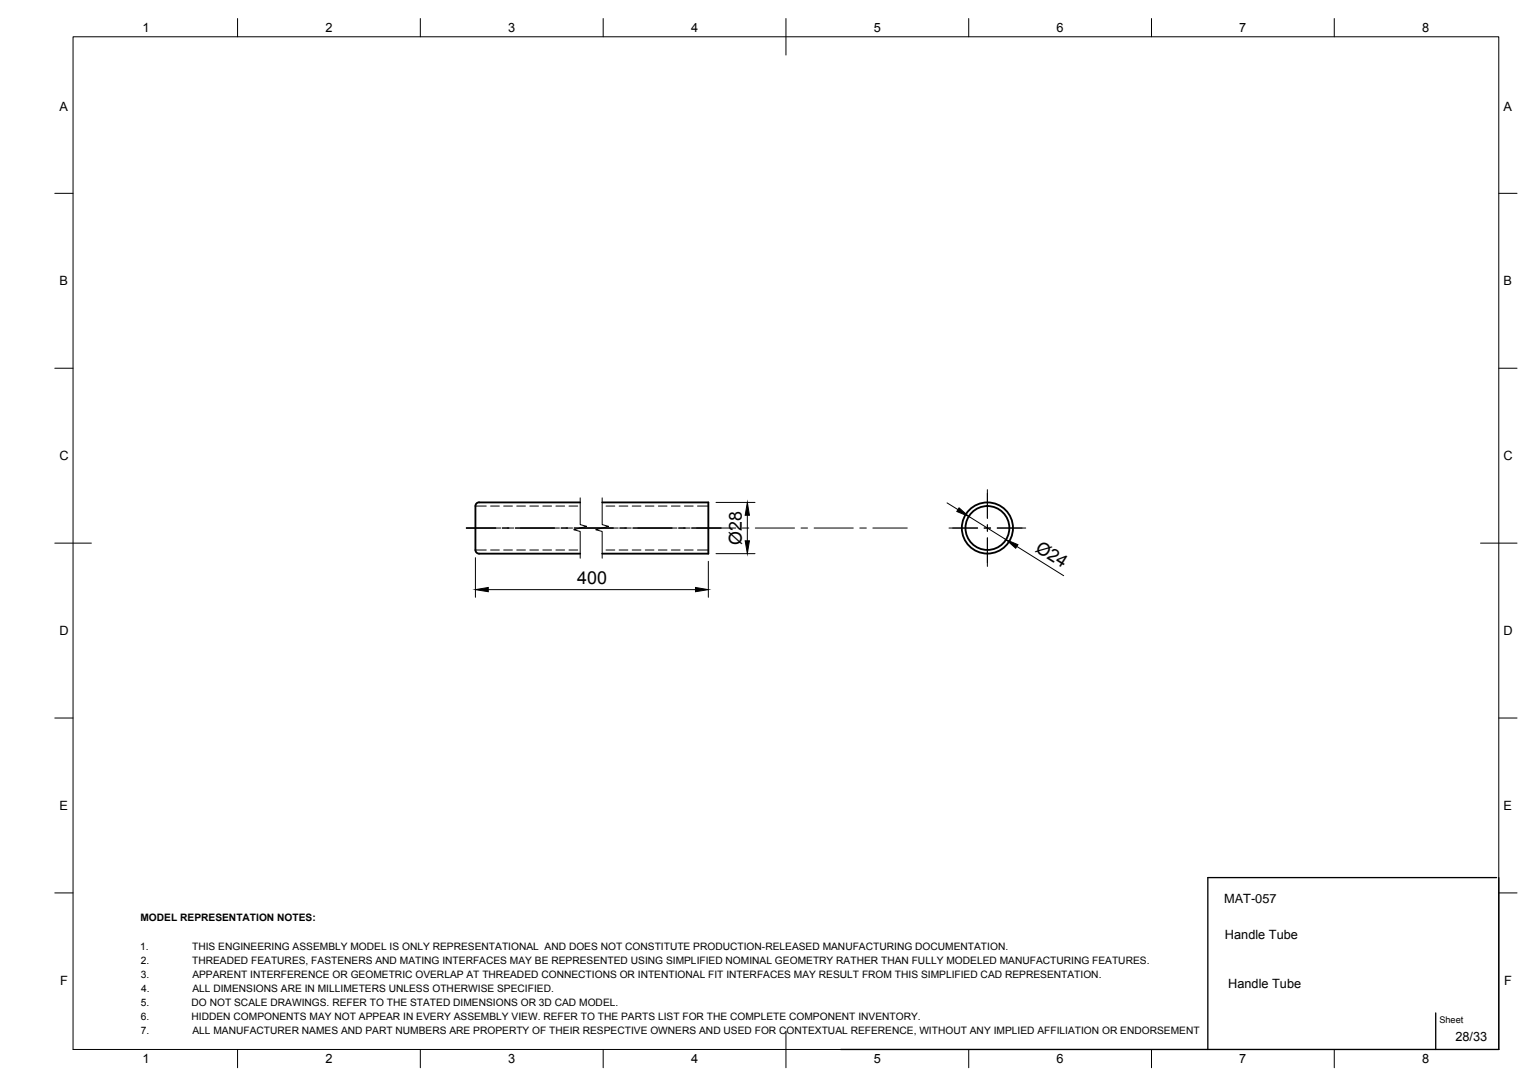
ISO-10303-21;
HEADER;
/* Generated by software containing ST-Developer
 * from STEP Tools, Inc. (www.steptools.com) 
 */

FILE_DESCRIPTION(
/* description */ ('STEP AP214', 'CAx-IF Rec.Pracs.---Representation and Presentation of Product Manufa
cturing Information (PMI)---4.0---2014-10-13'),
/* implementation_level */ '2;1');

FILE_NAME(
/* name */ 'Handle Tube.step',
/* time_stamp */ '2026-10-28T23:34:22+01:00',
/* author */ (''),
/* organization */ (''),
/* preprocessor_version */ 'ST-DEVELOPER v20.2',
/* originating_system */ 'Autodesk Translation Framework v15.17.0.0',
/* authorisation */ '');

FILE_SCHEMA (('AP242_MANAGED_MODEL_BASED_3D_ENGINEERING_MIM_LF { 1 0 10303 442 2 1 4 }'));
ENDSEC;

DATA;
#10=MECHANICAL_DESIGN_GEOMETRIC_PRESENTATION_REPRESENTATION('',(#269),#27807);
#221=SHAPE_REPRESENTATION_RELATIONSHIP('SRR','None',#27919,#243);
#243=ADVANCED_BREP_SHAPE_REPRESENTATION('',(#298),#27799);
#269=STYLED_ITEM('',(#28063),#298);
#298=MANIFOLD_SOLID_BREP('Body1',#12045);
#425=FACE_BOUND('',#2573,.T.);
#689=PLANE('',#13433);
#839=TOROIDAL_SURFACE('',#13423,12.,2.);
#1175=CYLINDRICAL_SURFACE('',#13429,12.);
#1176=CYLINDRICAL_SURFACE('',#13431,14.);
#1782=FACE_OUTER_BOUND('',#2569,.T.);
#1783=FACE_OUTER_BOUND('',#2570,.T.);
#1784=FACE_OUTER_BOUND('',#2571,.T.);
#1785=FACE_OUTER_BOUND('',#2572,.T.);
#2569=EDGE_LOOP('',(#10521,#10522,#10523,#10524,#10525,#10526));
#2570=EDGE_LOOP('',(#10527,#10528,#10529,#10530,#10531));
#2571=EDGE_LOOP('',(#10532,#10533,#10534,#10535,#10536));
#2572=EDGE_LOOP('',(#10537));
#2573=EDGE_LOOP('',(#10538));
#3418=LINE('',#23176,#4238);
#3419=LINE('',#23181,#4239);
#4238=VECTOR('',#16660,12.);
#4239=VECTOR('',#16667,14.);
#4918=CIRCLE('',#13424,12.);
#4919=CIRCLE('',#13425,12.);
#4920=CIRCLE('',#13426,2.);
#4921=CIRCLE('',#13427,14.);
#4922=CIRCLE('',#13428,14.);
#4923=CIRCLE('',#13430,12.);
#4924=CIRCLE('',#13432,14.);
#5891=VERTEX_POINT('',#23165);
#5892=VERTEX_POINT('',#23166);
#5893=VERTEX_POINT('',#23169);
#5894=VERTEX_POINT('',#23171);
#5895=VERTEX_POINT('',#23175);
#5896=VERTEX_POINT('',#23179);
#7473=EDGE_CURVE('',#5891,#5892,#4918,.T.);
#7474=EDGE_CURVE('',#5892,#5891,#4919,.T.);
#7475=EDGE_CURVE('',#5892,#5893,#4920,.T.);
#7476=EDGE_CURVE('',#5894,#5893,#4921,.T.);
#7477=EDGE_CURVE('',#5893,#5894,#4922,.T.);
#7478=EDGE_CURVE('',#5891,#5895,#3418,.T.);
#7479=EDGE_CURVE('',#5895,#5895,#4923,.T.);
#7480=EDGE_CURVE('',#5896,#5896,#4924,.T.);
#7481=EDGE_CURVE('',#5896,#5894,#3419,.T.);
#10521=ORIENTED_EDGE('',*,*,#7473,.F.);
#10522=ORIENTED_EDGE('',*,*,#7474,.F.);
#10523=ORIENTED_EDGE('',*,*,#7475,.T.);
#10524=ORIENTED_EDGE('',*,*,#7476,.F.);
#10525=ORIENTED_EDGE('',*,*,#7477,.F.);
#10526=ORIENTED_EDGE('',*,*,#7475,.F.);
#10527=ORIENTED_EDGE('',*,*,#7473,.T.);
#10528=ORIENTED_EDGE('',*,*,#7474,.T.);
#10529=ORIENTED_EDGE('',*,*,#7478,.T.);
#10530=ORIENTED_EDGE('',*,*,#7479,.F.);
#10531=ORIENTED_EDGE('',*,*,#7478,.F.);
#10532=ORIENTED_EDGE('',*,*,#7480,.T.);
#10533=ORIENTED_EDGE('',*,*,#7481,.T.);
#10534=ORIENTED_EDGE('',*,*,#7476,.T.);
#10535=ORIENTED_EDGE('',*,*,#7477,.T.);
#10536=ORIENTED_EDGE('',*,*,#7481,.F.);
#10537=ORIENTED_EDGE('',*,*,#7480,.F.);
#10538=ORIENTED_EDGE('',*,*,#7479,.T.);
#11864=ADVANCED_FACE('',(#1782),#839,.T.);
#11865=ADVANCED_FACE('',(#1783),#1175,.F.);
#11866=ADVANCED_FACE('',(#1784),#1176,.T.);
#11867=ADVANCED_FACE('',(#1785,#425),#689,.F.);
#12045=CLOSED_SHELL('',(#11864,#11865,#11866,#11867));
#13422=AXIS2_PLACEMENT_3D('',#23163,#16644,#16645);
#13423=AXIS2_PLACEMENT_3D('',#23164,#16646,#16647);
#13424=AXIS2_PLACEMENT_3D('',#23167,#16648,#16649);
#13425=AXIS2_PLACEMENT_3D('',#23168,#16650,#16651);
#13426=AXIS2_PLACEMENT_3D('',#23170,#16652,#16653);
#13427=AXIS2_PLACEMENT_3D('',#23172,#16654,#16655);
#13428=AXIS2_PLACEMENT_3D('',#23173,#16656,#16657);
#13429=AXIS2_PLACEMENT_3D('',#23174,#16658,#16659);
#13430=AXIS2_PLACEMENT_3D('',#23177,#16661,#16662);
#13431=AXIS2_PLACEMENT_3D('',#23178,#16663,#16664);
#13432=AXIS2_PLACEMENT_3D('',#23180,#16665,#16666);
#13433=AXIS2_PLACEMENT_3D('',#23182,#16668,#16669);
#16644=DIRECTION('axis',(0.,0.,1.));
#16645=DIRECTION('refdir',(1.,0.,0.));
#16646=DIRECTION('center_axis',(0.852431871234063,0.522838316216777,2.44136686633116E-17));
#16647=DIRECTION('ref_axis',(0.522838316216774,-0.852431871234064,0.));
#16648=DIRECTION('center_axis',(0.852431871234063,0.522838316216777,2.44136686633116E-17));
#16649=DIRECTION('ref_axis',(0.522838316216777,-0.852431871234063,8.32001735975286E-32));
#16650=DIRECTION('center_axis',(0.852431871234063,0.522838316216777,2.44136686633116E-17));
#16651=DIRECTION('ref_axis',(0.522838316216777,-0.852431871234063,8.32001735975286E-32));
#16652=DIRECTION('center_axis',(-2.08109892623551E-17,-1.27644014166001E-17,
1.));
#16653=DIRECTION('ref_axis',(-0.522838316216777,0.852431871234063,0.));
#16654=DIRECTION('center_axis',(-0.852431871234063,-0.522838316216777,-2.44136686633116E-17));
#16655=DIRECTION('ref_axis',(0.522838316216777,-0.852431871234063,1.54074395550979E-32));
#16656=DIRECTION('center_axis',(-0.852431871234063,-0.522838316216777,-2.44136686633116E-17));
#16657=DIRECTION('ref_axis',(0.522838316216777,-0.852431871234063,1.54074395550979E-32));
#16658=DIRECTION('center_axis',(-0.852431871234063,-0.522838316216777,-2.44136686633116E-17));
#16659=DIRECTION('ref_axis',(-0.522838316216777,0.852431871234063,-8.32001735975286E-32));
#16660=DIRECTION('',(-0.852431871234063,-0.522838316216777,-2.44136686633116E-17));
#16661=DIRECTION('center_axis',(0.852431871234063,0.522838316216777,2.44136686633116E-17));
#16662=DIRECTION('ref_axis',(0.522838316216777,-0.852431871234063,-1.54074395550979E-32));
#16663=DIRECTION('center_axis',(-0.852431871234063,-0.522838316216777,-2.44136686633116E-17));
#16664=DIRECTION('ref_axis',(-0.522838316216777,0.852431871234063,-1.54074395550979E-32));
#16665=DIRECTION('center_axis',(0.852431871234063,0.522838316216777,2.44136686633116E-17));
#16666=DIRECTION('ref_axis',(0.522838316216777,-0.852431871234063,1.54074395550979E-32));
#16667=DIRECTION('',(0.852431871234063,0.522838316216777,2.44136686633116E-17));
#16668=DIRECTION('center_axis',(0.852431871234063,0.522838316216777,2.44136686633116E-17));
#16669=DIRECTION('ref_axis',(0.522838316216777,-0.852431871234063,-1.10549867763274E-16));
#23163=CARTESIAN_POINT('',(0.,0.,0.));
#23164=CARTESIAN_POINT('Origin',(636.476617503915,410.22947428139,260.073593133703));
#23165=CARTESIAN_POINT('',(644.455541040985,401.045968459015,260.073593133703));
#23166=CARTESIAN_POINT('',(631.907421451782,421.504333368632,260.073593133703));
#23167=CARTESIAN_POINT('Origin',(638.181481246383,411.275150913823,260.073593133703));
#23168=CARTESIAN_POINT('Origin',(638.181481246383,411.275150913823,260.073593133703));
#23169=CARTESIAN_POINT('',(629.15688107688,422.163520478667,260.073593133703));
#23170=CARTESIAN_POINT('Origin',(630.202557709314,420.458656736199,260.073593133703));
#23171=CARTESIAN_POINT('',(643.79635393095,398.295428084113,260.073593133703));
#23172=CARTESIAN_POINT('Origin',(636.476617503915,410.22947428139,260.073593133703));
#23173=CARTESIAN_POINT('Origin',(636.476617503915,410.22947428139,260.073593133703));
#23174=CARTESIAN_POINT('Origin',(638.181481246383,411.275150913823,260.073593133703));
#23175=CARTESIAN_POINT('',(303.482792547359,191.910641972304,260.073593133703));
#23176=CARTESIAN_POINT('',(644.455541040985,401.045968459015,260.073593133703));
#23177=CARTESIAN_POINT('Origin',(297.208732752758,202.139824427113,260.073593133703));
#23178=CARTESIAN_POINT('Origin',(638.181481246383,411.275150913823,260.073593133703));
#23179=CARTESIAN_POINT('',(304.528469179793,190.205778229836,260.073593133703));
#23180=CARTESIAN_POINT('Origin',(297.208732752758,202.139824427113,260.073593133703));
#23181=CARTESIAN_POINT('',(645.501217673418,399.341104716547,260.073593133703));
#23182=CARTESIAN_POINT('Origin',(297.208732752758,202.139824427113,260.073593133703));
#27770=UNCERTAINTY_MEASURE_WITH_UNIT(LENGTH_MEASURE(0.01),#27808,
'DISTANCE_ACCURACY_VALUE',
'Maximum model space distance between geometric entities at asserted c
onnectivities');
#27778=UNCERTAINTY_MEASURE_WITH_UNIT(LENGTH_MEASURE(0.01),#27808,
'DISTANCE_ACCURACY_VALUE',
'Maximum model space distance between geometric entities at asserted c
onnectivities');
#27799=(
GEOMETRIC_REPRESENTATION_CONTEXT(3)
GLOBAL_UNCERTAINTY_ASSIGNED_CONTEXT((#27770))
GLOBAL_UNIT_ASSIGNED_CONTEXT((#27808,#27810,#27811))
REPRESENTATION_CONTEXT('','3D')
);
#27807=(
GEOMETRIC_REPRESENTATION_CONTEXT(3)
GLOBAL_UNCERTAINTY_ASSIGNED_CONTEXT((#27778))
GLOBAL_UNIT_ASSIGNED_CONTEXT((#27808,#27810,#27811))
REPRESENTATION_CONTEXT('','3D')
);
#27808=(
LENGTH_UNIT()
NAMED_UNIT(*)
SI_UNIT(.MILLI.,.METRE.)
);
#27810=(
NAMED_UNIT(*)
PLANE_ANGLE_UNIT()
SI_UNIT($,.RADIAN.)
);
#27811=(
NAMED_UNIT(*)
SI_UNIT($,.STERADIAN.)
SOLID_ANGLE_UNIT()
);
#27832=SHAPE_DEFINITION_REPRESENTATION(#27872,#27919);
#27872=PRODUCT_DEFINITION_SHAPE('',$,#27948);
#27919=SHAPE_REPRESENTATION('',(#13422),#27799);
#27927=PRODUCT_DEFINITION_CONTEXT('part definition',#28013,'design');
#27948=PRODUCT_DEFINITION('Handle Tube','Handle Tube',#27976,#27927);
#27976=PRODUCT_DEFINITION_FORMATION('',$,#28035);
#28013=APPLICATION_CONTEXT('Managed model based 3d engineering');
#28014=PRODUCT_CONTEXT('part definition',#28013,'mechanical');
#28035=PRODUCT('Handle Tube','Handle Tube',$,(#28014));
#28057=COLOUR_RGB('Light Blue',0.38,0.62,0.78);
#28058=FILL_AREA_STYLE_COLOUR('',#28057);
#28059=FILL_AREA_STYLE('',(#28058));
#28060=SURFACE_STYLE_FILL_AREA(#28059);
#28061=SURFACE_SIDE_STYLE('',(#28060));
#28062=SURFACE_STYLE_USAGE(.BOTH.,#28061);
#28063=PRESENTATION_STYLE_ASSIGNMENT((#28062));
ENDSEC;
END-ISO-10303-21;
